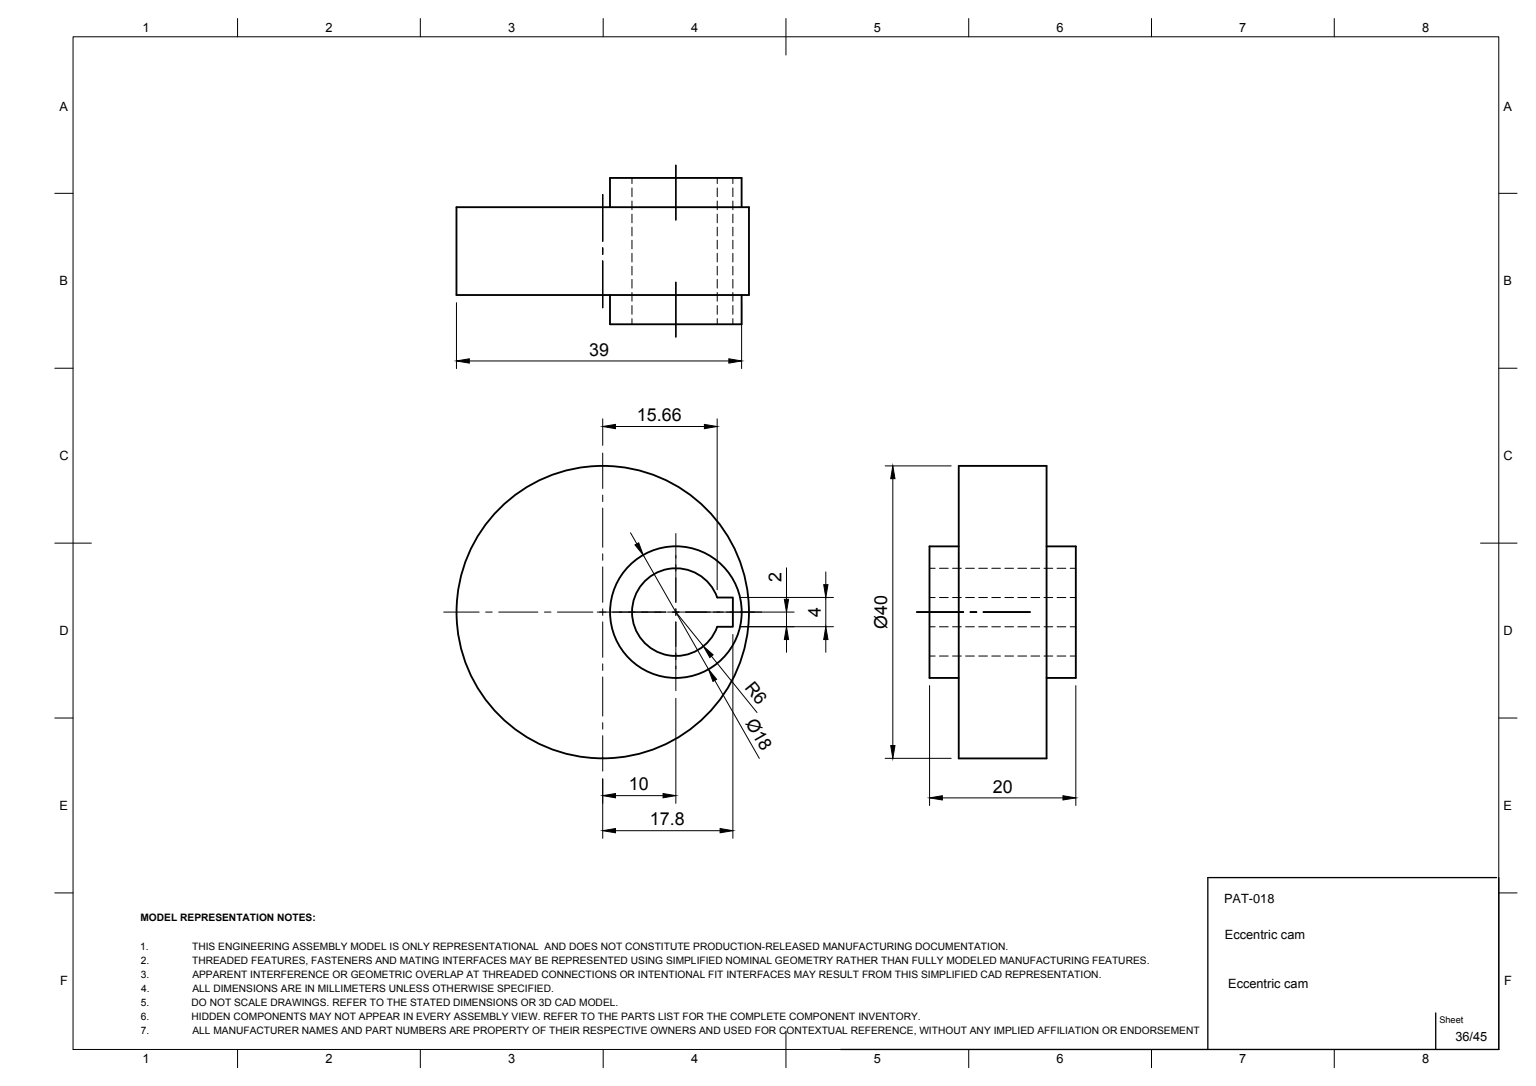
ISO-10303-21;
HEADER;
/* Generated by software containing ST-Developer
 * from STEP Tools, Inc. (www.steptools.com) 
 */

FILE_DESCRIPTION(
/* description */ ('Cam-driven reciprocating slide'),
/* implementation_level */ '2;1');

FILE_NAME(
/* name */ 'Eccentric cam.step',
/* time_stamp */ '2026-10-28T03:25:20-07:00',
/* author */ (''),
/* organization */ (''),
/* preprocessor_version */ 'ST-DEVELOPER v20.2',
/* originating_system */ 'Autodesk Translation Framework v15.17.0.0',
/* authorisation */ '');

FILE_SCHEMA (('AUTOMOTIVE_DESIGN { 1 0 10303 214 3 1 1 }'));
ENDSEC;

DATA;
#10=MECHANICAL_DESIGN_GEOMETRIC_PRESENTATION_REPRESENTATION('',(#456),#13277);
#375=SHAPE_REPRESENTATION_RELATIONSHIP('SRR','None',#13471,#412);
#412=ADVANCED_BREP_SHAPE_REPRESENTATION('',(#498),#13266);
#456=STYLED_ITEM('',(#13734),#498);
#498=MANIFOLD_SOLID_BREP('Body2',#6434);
#652=FACE_BOUND('',#1719,.T.);
#653=FACE_BOUND('',#1724,.T.);
#654=FACE_BOUND('',#1727,.T.);
#655=FACE_BOUND('',#1729,.T.);
#841=PLANE('',#7450);
#842=PLANE('',#7451);
#843=PLANE('',#7452);
#844=PLANE('',#7453);
#845=PLANE('',#7463);
#846=PLANE('',#7467);
#847=PLANE('',#7468);
#1191=FACE_OUTER_BOUND('',#1715,.T.);
#1192=FACE_OUTER_BOUND('',#1716,.T.);
#1193=FACE_OUTER_BOUND('',#1717,.T.);
#1194=FACE_OUTER_BOUND('',#1718,.T.);
#1195=FACE_OUTER_BOUND('',#1720,.T.);
#1196=FACE_OUTER_BOUND('',#1721,.T.);
#1197=FACE_OUTER_BOUND('',#1722,.T.);
#1198=FACE_OUTER_BOUND('',#1723,.T.);
#1199=FACE_OUTER_BOUND('',#1725,.T.);
#1200=FACE_OUTER_BOUND('',#1726,.T.);
#1201=FACE_OUTER_BOUND('',#1728,.T.);
#1715=EDGE_LOOP('',(#5540,#5541,#5542,#5543));
#1716=EDGE_LOOP('',(#5544,#5545,#5546,#5547));
#1717=EDGE_LOOP('',(#5548,#5549,#5550,#5551));
#1718=EDGE_LOOP('',(#5552));
#1719=EDGE_LOOP('',(#5553,#5554,#5555,#5556));
#1720=EDGE_LOOP('',(#5557,#5558,#5559,#5560));
#1721=EDGE_LOOP('',(#5561,#5562,#5563,#5564));
#1722=EDGE_LOOP('',(#5565,#5566,#5567,#5568));
#1723=EDGE_LOOP('',(#5569));
#1724=EDGE_LOOP('',(#5570,#5571,#5572,#5573));
#1725=EDGE_LOOP('',(#5574,#5575,#5576,#5577));
#1726=EDGE_LOOP('',(#5578));
#1727=EDGE_LOOP('',(#5579));
#1728=EDGE_LOOP('',(#5580));
#1729=EDGE_LOOP('',(#5581));
#2152=LINE('',#12738,#2591);
#2153=LINE('',#12740,#2592);
#2154=LINE('',#12742,#2593);
#2155=LINE('',#12743,#2594);
#2156=LINE('',#12746,#2595);
#2157=LINE('',#12748,#2596);
#2158=LINE('',#12749,#2597);
#2159=LINE('',#12752,#2598);
#2160=LINE('',#12754,#2599);
#2161=LINE('',#12755,#2600);
#2162=LINE('',#12766,#2601);
#2163=LINE('',#12770,#2602);
#2164=LINE('',#12777,#2603);
#2591=VECTOR('',#9184,1.);
#2592=VECTOR('',#9185,1.);
#2593=VECTOR('',#9186,1.);
#2594=VECTOR('',#9187,1.);
#2595=VECTOR('',#9190,1.);
#2596=VECTOR('',#9191,1.);
#2597=VECTOR('',#9192,1.);
#2598=VECTOR('',#9195,1.);
#2599=VECTOR('',#9196,1.);
#2600=VECTOR('',#9197,1.);
#2601=VECTOR('',#9212,0.9);
#2602=VECTOR('',#9217,0.9);
#2603=VECTOR('',#9226,2.);
#2979=CIRCLE('',#7454,0.9);
#2980=CIRCLE('',#7455,0.6);
#2981=CIRCLE('',#7457,0.6);
#2982=CIRCLE('',#7459,0.9);
#2983=CIRCLE('',#7460,0.9);
#2984=CIRCLE('',#7462,0.9);
#2985=CIRCLE('',#7465,2.);
#2986=CIRCLE('',#7466,2.);
#3442=VERTEX_POINT('',#12736);
#3443=VERTEX_POINT('',#12737);
#3444=VERTEX_POINT('',#12739);
#3445=VERTEX_POINT('',#12741);
#3446=VERTEX_POINT('',#12745);
#3447=VERTEX_POINT('',#12747);
#3448=VERTEX_POINT('',#12751);
#3449=VERTEX_POINT('',#12753);
#3450=VERTEX_POINT('',#12757);
#3451=VERTEX_POINT('',#12763);
#3452=VERTEX_POINT('',#12765);
#3453=VERTEX_POINT('',#12769);
#3454=VERTEX_POINT('',#12774);
#3455=VERTEX_POINT('',#12776);
#4160=EDGE_CURVE('',#3442,#3443,#2152,.T.);
#4161=EDGE_CURVE('',#3442,#3444,#2153,.T.);
#4162=EDGE_CURVE('',#3445,#3444,#2154,.T.);
#4163=EDGE_CURVE('',#3443,#3445,#2155,.T.);
#4164=EDGE_CURVE('',#3446,#3442,#2156,.T.);
#4165=EDGE_CURVE('',#3446,#3447,#2157,.T.);
#4166=EDGE_CURVE('',#3444,#3447,#2158,.T.);
#4167=EDGE_CURVE('',#3448,#3446,#2159,.T.);
#4168=EDGE_CURVE('',#3449,#3448,#2160,.T.);
#4169=EDGE_CURVE('',#3447,#3449,#2161,.T.);
#4170=EDGE_CURVE('',#3450,#3450,#2979,.T.);
#4171=EDGE_CURVE('',#3449,#3445,#2980,.T.);
#4172=EDGE_CURVE('',#3443,#3448,#2981,.T.);
#4173=EDGE_CURVE('',#3451,#3451,#2982,.T.);
#4174=EDGE_CURVE('',#3451,#3452,#2162,.T.);
#4175=EDGE_CURVE('',#3452,#3452,#2983,.T.);
#4176=EDGE_CURVE('',#3450,#3453,#2163,.T.);
#4177=EDGE_CURVE('',#3453,#3453,#2984,.T.);
#4178=EDGE_CURVE('',#3454,#3454,#2985,.T.);
#4179=EDGE_CURVE('',#3454,#3455,#2164,.T.);
#4180=EDGE_CURVE('',#3455,#3455,#2986,.T.);
#5540=ORIENTED_EDGE('',*,*,#4160,.F.);
#5541=ORIENTED_EDGE('',*,*,#4161,.T.);
#5542=ORIENTED_EDGE('',*,*,#4162,.F.);
#5543=ORIENTED_EDGE('',*,*,#4163,.F.);
#5544=ORIENTED_EDGE('',*,*,#4164,.F.);
#5545=ORIENTED_EDGE('',*,*,#4165,.T.);
#5546=ORIENTED_EDGE('',*,*,#4166,.F.);
#5547=ORIENTED_EDGE('',*,*,#4161,.F.);
#5548=ORIENTED_EDGE('',*,*,#4167,.F.);
#5549=ORIENTED_EDGE('',*,*,#4168,.F.);
#5550=ORIENTED_EDGE('',*,*,#4169,.F.);
#5551=ORIENTED_EDGE('',*,*,#4165,.F.);
#5552=ORIENTED_EDGE('',*,*,#4170,.T.);
#5553=ORIENTED_EDGE('',*,*,#4162,.T.);
#5554=ORIENTED_EDGE('',*,*,#4166,.T.);
#5555=ORIENTED_EDGE('',*,*,#4169,.T.);
#5556=ORIENTED_EDGE('',*,*,#4171,.T.);
#5557=ORIENTED_EDGE('',*,*,#4163,.T.);
#5558=ORIENTED_EDGE('',*,*,#4171,.F.);
#5559=ORIENTED_EDGE('',*,*,#4168,.T.);
#5560=ORIENTED_EDGE('',*,*,#4172,.F.);
#5561=ORIENTED_EDGE('',*,*,#4173,.F.);
#5562=ORIENTED_EDGE('',*,*,#4174,.T.);
#5563=ORIENTED_EDGE('',*,*,#4175,.T.);
#5564=ORIENTED_EDGE('',*,*,#4174,.F.);
#5565=ORIENTED_EDGE('',*,*,#4170,.F.);
#5566=ORIENTED_EDGE('',*,*,#4176,.T.);
#5567=ORIENTED_EDGE('',*,*,#4177,.F.);
#5568=ORIENTED_EDGE('',*,*,#4176,.F.);
#5569=ORIENTED_EDGE('',*,*,#4175,.F.);
#5570=ORIENTED_EDGE('',*,*,#4160,.T.);
#5571=ORIENTED_EDGE('',*,*,#4172,.T.);
#5572=ORIENTED_EDGE('',*,*,#4167,.T.);
#5573=ORIENTED_EDGE('',*,*,#4164,.T.);
#5574=ORIENTED_EDGE('',*,*,#4178,.F.);
#5575=ORIENTED_EDGE('',*,*,#4179,.T.);
#5576=ORIENTED_EDGE('',*,*,#4180,.T.);
#5577=ORIENTED_EDGE('',*,*,#4179,.F.);
#5578=ORIENTED_EDGE('',*,*,#4178,.T.);
#5579=ORIENTED_EDGE('',*,*,#4177,.T.);
#5580=ORIENTED_EDGE('',*,*,#4180,.F.);
#5581=ORIENTED_EDGE('',*,*,#4173,.T.);
#5994=CYLINDRICAL_SURFACE('',#7456,0.6);
#5995=CYLINDRICAL_SURFACE('',#7458,0.9);
#5996=CYLINDRICAL_SURFACE('',#7461,0.9);
#5997=CYLINDRICAL_SURFACE('',#7464,2.);
#6309=ADVANCED_FACE('',(#1191),#841,.F.);
#6310=ADVANCED_FACE('',(#1192),#842,.F.);
#6311=ADVANCED_FACE('',(#1193),#843,.F.);
#6312=ADVANCED_FACE('',(#1194,#652),#844,.T.);
#6313=ADVANCED_FACE('',(#1195),#5994,.F.);
#6314=ADVANCED_FACE('',(#1196),#5995,.T.);
#6315=ADVANCED_FACE('',(#1197),#5996,.T.);
#6316=ADVANCED_FACE('',(#1198,#653),#845,.F.);
#6317=ADVANCED_FACE('',(#1199),#5997,.T.);
#6318=ADVANCED_FACE('',(#1200,#654),#846,.T.);
#6319=ADVANCED_FACE('',(#1201,#655),#847,.F.);
#6434=CLOSED_SHELL('',(#6309,#6310,#6311,#6312,#6313,#6314,#6315,#6316,
#6317,#6318,#6319));
#7449=AXIS2_PLACEMENT_3D('',#12734,#9180,#9181);
#7450=AXIS2_PLACEMENT_3D('',#12735,#9182,#9183);
#7451=AXIS2_PLACEMENT_3D('',#12744,#9188,#9189);
#7452=AXIS2_PLACEMENT_3D('',#12750,#9193,#9194);
#7453=AXIS2_PLACEMENT_3D('',#12756,#9198,#9199);
#7454=AXIS2_PLACEMENT_3D('',#12758,#9200,#9201);
#7455=AXIS2_PLACEMENT_3D('',#12759,#9202,#9203);
#7456=AXIS2_PLACEMENT_3D('',#12760,#9204,#9205);
#7457=AXIS2_PLACEMENT_3D('',#12761,#9206,#9207);
#7458=AXIS2_PLACEMENT_3D('',#12762,#9208,#9209);
#7459=AXIS2_PLACEMENT_3D('',#12764,#9210,#9211);
#7460=AXIS2_PLACEMENT_3D('',#12767,#9213,#9214);
#7461=AXIS2_PLACEMENT_3D('',#12768,#9215,#9216);
#7462=AXIS2_PLACEMENT_3D('',#12771,#9218,#9219);
#7463=AXIS2_PLACEMENT_3D('',#12772,#9220,#9221);
#7464=AXIS2_PLACEMENT_3D('',#12773,#9222,#9223);
#7465=AXIS2_PLACEMENT_3D('',#12775,#9224,#9225);
#7466=AXIS2_PLACEMENT_3D('',#12778,#9227,#9228);
#7467=AXIS2_PLACEMENT_3D('',#12779,#9229,#9230);
#7468=AXIS2_PLACEMENT_3D('',#12780,#9231,#9232);
#9180=DIRECTION('axis',(0.,0.,1.));
#9181=DIRECTION('refdir',(1.,0.,0.));
#9182=DIRECTION('center_axis',(-1.,0.,0.));
#9183=DIRECTION('ref_axis',(0.,0.,1.));
#9184=DIRECTION('',(0.,0.,1.));
#9185=DIRECTION('',(0.,1.,0.));
#9186=DIRECTION('',(0.,0.,-1.));
#9187=DIRECTION('',(0.,1.,0.));
#9188=DIRECTION('center_axis',(0.,0.,-1.));
#9189=DIRECTION('ref_axis',(-1.,0.,0.));
#9190=DIRECTION('',(-1.,0.,0.));
#9191=DIRECTION('',(0.,1.,0.));
#9192=DIRECTION('',(1.,0.,0.));
#9193=DIRECTION('center_axis',(1.,0.,0.));
#9194=DIRECTION('ref_axis',(0.,0.,-1.));
#9195=DIRECTION('',(0.,0.,-1.));
#9196=DIRECTION('',(0.,-1.,0.));
#9197=DIRECTION('',(0.,0.,1.));
#9198=DIRECTION('center_axis',(0.,1.,0.));
#9199=DIRECTION('ref_axis',(1.,0.,0.));
#9200=DIRECTION('center_axis',(0.,1.,0.));
#9201=DIRECTION('ref_axis',(1.,0.,0.));
#9202=DIRECTION('center_axis',(0.,-1.,0.));
#9203=DIRECTION('ref_axis',(1.,0.,0.));
#9204=DIRECTION('center_axis',(0.,1.,0.));
#9205=DIRECTION('ref_axis',(-1.83697019872103E-16,0.,1.));
#9206=DIRECTION('center_axis',(0.,1.,0.));
#9207=DIRECTION('ref_axis',(1.,0.,0.));
#9208=DIRECTION('center_axis',(0.,1.,0.));
#9209=DIRECTION('ref_axis',(1.,0.,0.));
#9210=DIRECTION('center_axis',(0.,1.,0.));
#9211=DIRECTION('ref_axis',(1.,0.,0.));
#9212=DIRECTION('',(0.,-1.,0.));
#9213=DIRECTION('center_axis',(0.,1.,0.));
#9214=DIRECTION('ref_axis',(1.,0.,0.));
#9215=DIRECTION('center_axis',(0.,1.,0.));
#9216=DIRECTION('ref_axis',(1.,0.,0.));
#9217=DIRECTION('',(0.,-1.,0.));
#9218=DIRECTION('center_axis',(0.,-1.,0.));
#9219=DIRECTION('ref_axis',(1.,0.,0.));
#9220=DIRECTION('center_axis',(0.,1.,0.));
#9221=DIRECTION('ref_axis',(1.,0.,0.));
#9222=DIRECTION('center_axis',(0.,1.,0.));
#9223=DIRECTION('ref_axis',(1.,0.,0.));
#9224=DIRECTION('center_axis',(0.,1.,0.));
#9225=DIRECTION('ref_axis',(1.,0.,0.));
#9226=DIRECTION('',(0.,-1.,0.));
#9227=DIRECTION('center_axis',(0.,1.,0.));
#9228=DIRECTION('ref_axis',(1.,0.,0.));
#9229=DIRECTION('center_axis',(0.,1.,0.));
#9230=DIRECTION('ref_axis',(1.,0.,0.));
#9231=DIRECTION('center_axis',(0.,1.,0.));
#9232=DIRECTION('ref_axis',(1.,0.,0.));
#12734=CARTESIAN_POINT('',(0.,0.,0.));
#12735=CARTESIAN_POINT('Origin',(-0.2,-1.1,3.22));
#12736=CARTESIAN_POINT('',(-0.2,-1.,3.22));
#12737=CARTESIAN_POINT('',(-0.2,-1.,3.43431457505076));
#12738=CARTESIAN_POINT('',(-0.2,-1.,3.61));
#12739=CARTESIAN_POINT('',(-0.2,1.,3.22));
#12740=CARTESIAN_POINT('',(-0.2,-1.1,3.22));
#12741=CARTESIAN_POINT('',(-0.2,1.,3.43431457505076));
#12742=CARTESIAN_POINT('',(-0.2,1.,3.61));
#12743=CARTESIAN_POINT('',(-0.2,-1.1,3.43431457505076));
#12744=CARTESIAN_POINT('Origin',(0.2,-1.1,3.22));
#12745=CARTESIAN_POINT('',(0.2,-1.,3.22));
#12746=CARTESIAN_POINT('',(0.1,-1.,3.22));
#12747=CARTESIAN_POINT('',(0.2,1.,3.22));
#12748=CARTESIAN_POINT('',(0.2,-1.1,3.22));
#12749=CARTESIAN_POINT('',(0.1,1.,3.22));
#12750=CARTESIAN_POINT('Origin',(0.2,-1.1,4.));
#12751=CARTESIAN_POINT('',(0.2,-1.,3.43431457505076));
#12752=CARTESIAN_POINT('',(0.2,-1.,4.));
#12753=CARTESIAN_POINT('',(0.2,1.,3.43431457505076));
#12754=CARTESIAN_POINT('',(0.2,-1.1,3.43431457505076));
#12755=CARTESIAN_POINT('',(0.2,1.,4.));
#12756=CARTESIAN_POINT('Origin',(0.,1.,4.));
#12757=CARTESIAN_POINT('',(-0.9,1.,4.));
#12758=CARTESIAN_POINT('Origin',(0.,1.,4.));
#12759=CARTESIAN_POINT('Origin',(0.,1.,4.));
#12760=CARTESIAN_POINT('Origin',(0.,-1.1,4.));
#12761=CARTESIAN_POINT('Origin',(0.,-1.,4.));
#12762=CARTESIAN_POINT('Origin',(0.,-1.,4.));
#12763=CARTESIAN_POINT('',(-0.9,-0.6,4.));
#12764=CARTESIAN_POINT('Origin',(0.,-0.6,4.));
#12765=CARTESIAN_POINT('',(-0.9,-1.,4.));
#12766=CARTESIAN_POINT('',(-0.9,-1.,4.));
#12767=CARTESIAN_POINT('Origin',(0.,-1.,4.));
#12768=CARTESIAN_POINT('Origin',(0.,-1.,4.));
#12769=CARTESIAN_POINT('',(-0.9,0.6,4.));
#12770=CARTESIAN_POINT('',(-0.9,-1.,4.));
#12771=CARTESIAN_POINT('Origin',(0.,0.6,4.));
#12772=CARTESIAN_POINT('Origin',(0.,-1.,4.));
#12773=CARTESIAN_POINT('Origin',(0.,-0.6,5.));
#12774=CARTESIAN_POINT('',(-2.,0.6,5.));
#12775=CARTESIAN_POINT('Origin',(0.,0.6,5.));
#12776=CARTESIAN_POINT('',(-2.,-0.6,5.));
#12777=CARTESIAN_POINT('',(-2.,-0.6,5.));
#12778=CARTESIAN_POINT('Origin',(0.,-0.6,5.));
#12779=CARTESIAN_POINT('Origin',(0.,0.6,5.));
#12780=CARTESIAN_POINT('Origin',(0.,-0.6,5.));
#13222=UNCERTAINTY_MEASURE_WITH_UNIT(LENGTH_MEASURE(0.001),#13278,
'DISTANCE_ACCURACY_VALUE',
'Maximum model space distance between geometric entities at asserted c
onnectivities');
#13233=UNCERTAINTY_MEASURE_WITH_UNIT(LENGTH_MEASURE(0.001),#13278,
'DISTANCE_ACCURACY_VALUE',
'Maximum model space distance between geometric entities at asserted c
onnectivities');
#13266=(
GEOMETRIC_REPRESENTATION_CONTEXT(3)
GLOBAL_UNCERTAINTY_ASSIGNED_CONTEXT((#13222))
GLOBAL_UNIT_ASSIGNED_CONTEXT((#13278,#13280,#13281))
REPRESENTATION_CONTEXT('','3D')
);
#13277=(
GEOMETRIC_REPRESENTATION_CONTEXT(3)
GLOBAL_UNCERTAINTY_ASSIGNED_CONTEXT((#13233))
GLOBAL_UNIT_ASSIGNED_CONTEXT((#13278,#13280,#13281))
REPRESENTATION_CONTEXT('','3D')
);
#13278=(
LENGTH_UNIT()
NAMED_UNIT(*)
SI_UNIT(.CENTI.,.METRE.)
);
#13280=(
NAMED_UNIT(*)
PLANE_ANGLE_UNIT()
SI_UNIT($,.RADIAN.)
);
#13281=(
NAMED_UNIT(*)
SI_UNIT($,.STERADIAN.)
SOLID_ANGLE_UNIT()
);
#13314=SHAPE_DEFINITION_REPRESENTATION(#13364,#13471);
#13364=PRODUCT_DEFINITION_SHAPE('',$,#13515);
#13471=SHAPE_REPRESENTATION('',(#7449),#13266);
#13482=PRODUCT_DEFINITION_CONTEXT('part definition',#13613,'design');
#13515=PRODUCT_DEFINITION('Eccentric cam','Eccentric cam',#13558,#13482);
#13558=PRODUCT_DEFINITION_FORMATION('',$,#13647);
#13613=APPLICATION_CONTEXT(
'Core Data for Automotive Mechanical Design Process');
#13614=PRODUCT_CONTEXT('part definition',#13613,'mechanical');
#13647=PRODUCT('Eccentric cam','Eccentric cam','Eccentric cam',(#13614));
#13728=COLOUR_RGB('Off White',0.89,0.88,0.83);
#13729=FILL_AREA_STYLE_COLOUR('',#13728);
#13730=FILL_AREA_STYLE('',(#13729));
#13731=SURFACE_STYLE_FILL_AREA(#13730);
#13732=SURFACE_SIDE_STYLE('',(#13731));
#13733=SURFACE_STYLE_USAGE(.BOTH.,#13732);
#13734=PRESENTATION_STYLE_ASSIGNMENT((#13733));
ENDSEC;
END-ISO-10303-21;
